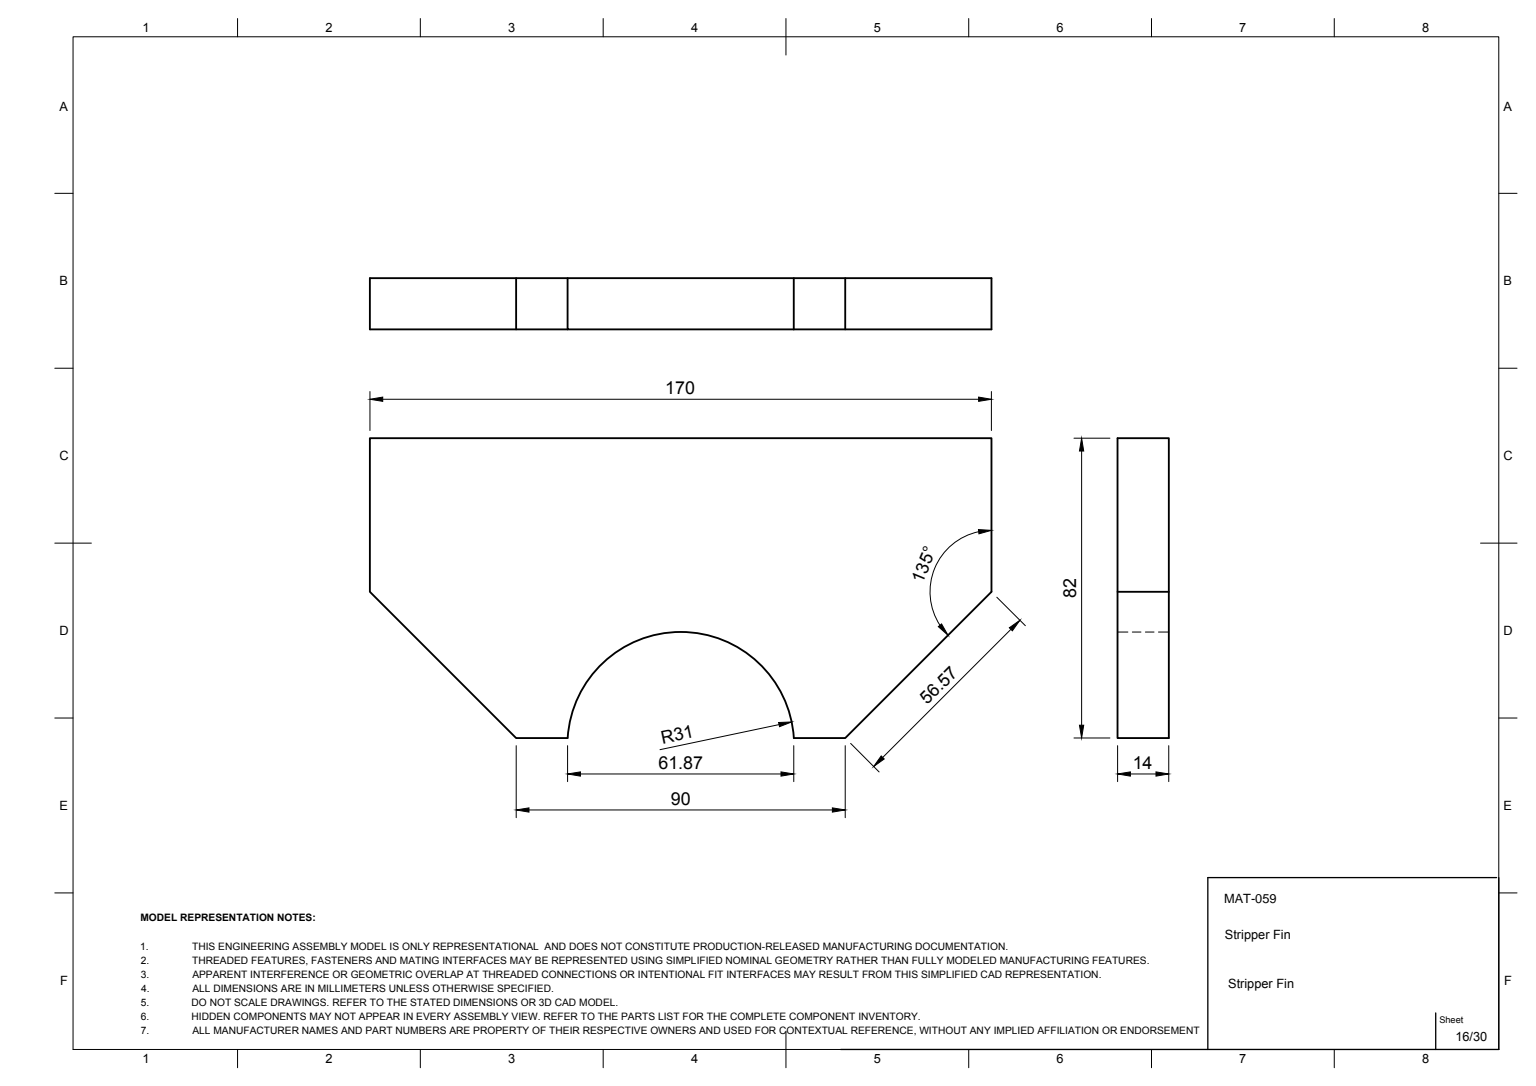
ISO-10303-21;
HEADER;
/* Generated by software containing ST-Developer
 * from STEP Tools, Inc. (www.steptools.com) 
 */

FILE_DESCRIPTION(
/* description */ ('', 'CAx-IF Rec.Pracs.---Representation and Presentation of Product Manufa
cturing Information (PMI)---4.0---2014-10-13'),
/* implementation_level */ '2;1');

FILE_NAME(
/* name */ 'Stripper Fin.step',
/* time_stamp */ '2026-10-28T23:00:48+01:00',
/* author */ (''),
/* organization */ (''),
/* preprocessor_version */ 'ST-DEVELOPER v20.2',
/* originating_system */ 'Autodesk Translation Framework v15.17.0.0',
/* authorisation */ '');

FILE_SCHEMA (('AP242_MANAGED_MODEL_BASED_3D_ENGINEERING_MIM_LF { 1 0 10303 442 2 1 4 }'));
ENDSEC;

DATA;
#10=MECHANICAL_DESIGN_GEOMETRIC_PRESENTATION_REPRESENTATION('',(#990),#61811);
#926=SHAPE_REPRESENTATION_RELATIONSHIP('SRR','None',#61985,#951);
#951=ADVANCED_BREP_SHAPE_REPRESENTATION('',(#1029),#61798);
#990=STYLED_ITEM('',(#62142),#1029);
#1029=MANIFOLD_SOLID_BREP('Body1',#33820);
#1365=CYLINDRICAL_SURFACE('',#35914,31.);
#3028=CIRCLE('',#35913,31.);
#3029=CIRCLE('',#35915,31.);
#5170=FACE_OUTER_BOUND('',#7276,.T.);
#5171=FACE_OUTER_BOUND('',#7277,.T.);
#5172=FACE_OUTER_BOUND('',#7278,.T.);
#5173=FACE_OUTER_BOUND('',#7279,.T.);
#5174=FACE_OUTER_BOUND('',#7280,.T.);
#5175=FACE_OUTER_BOUND('',#7281,.T.);
#5176=FACE_OUTER_BOUND('',#7282,.T.);
#5177=FACE_OUTER_BOUND('',#7283,.T.);
#5178=FACE_OUTER_BOUND('',#7284,.T.);
#5179=FACE_OUTER_BOUND('',#7285,.T.);
#7276=EDGE_LOOP('',(#26122,#26123,#26124,#26125));
#7277=EDGE_LOOP('',(#26126,#26127,#26128,#26129));
#7278=EDGE_LOOP('',(#26130,#26131,#26132,#26133,#26134,#26135,#26136,#26137));
#7279=EDGE_LOOP('',(#26138,#26139,#26140,#26141));
#7280=EDGE_LOOP('',(#26142,#26143,#26144,#26145,#26146,#26147,#26148,#26149));
#7281=EDGE_LOOP('',(#26150,#26151,#26152,#26153));
#7282=EDGE_LOOP('',(#26154,#26155,#26156,#26157));
#7283=EDGE_LOOP('',(#26158,#26159,#26160,#26161));
#7284=EDGE_LOOP('',(#26162,#26163,#26164,#26165));
#7285=EDGE_LOOP('',(#26166,#26167,#26168,#26169));
#9707=LINE('',#55749,#12254);
#9708=LINE('',#55751,#12255);
#9709=LINE('',#55753,#12256);
#9710=LINE('',#55754,#12257);
#9711=LINE('',#55757,#12258);
#9712=LINE('',#55759,#12259);
#9713=LINE('',#55760,#12260);
#9714=LINE('',#55763,#12261);
#9715=LINE('',#55765,#12262);
#9716=LINE('',#55767,#12263);
#9717=LINE('',#55771,#12264);
#9718=LINE('',#55772,#12265);
#9719=LINE('',#55775,#12266);
#9720=LINE('',#55777,#12267);
#9721=LINE('',#55781,#12268);
#9722=LINE('',#55782,#12269);
#9723=LINE('',#55784,#12270);
#9724=LINE('',#55786,#12271);
#9725=LINE('',#55787,#12272);
#9726=LINE('',#55789,#12273);
#9727=LINE('',#55791,#12274);
#9728=LINE('',#55793,#12275);
#12254=VECTOR('',#43125,10.);
#12255=VECTOR('',#43126,10.);
#12256=VECTOR('',#43127,10.);
#12257=VECTOR('',#43128,10.);
#12258=VECTOR('',#43131,10.);
#12259=VECTOR('',#43132,10.);
#12260=VECTOR('',#43133,10.);
#12261=VECTOR('',#43136,10.);
#12262=VECTOR('',#43137,10.);
#12263=VECTOR('',#43138,10.);
#12264=VECTOR('',#43141,10.);
#12265=VECTOR('',#43142,10.);
#12266=VECTOR('',#43145,10.);
#12267=VECTOR('',#43146,10.);
#12268=VECTOR('',#43151,10.);
#12269=VECTOR('',#43152,10.);
#12270=VECTOR('',#43153,10.);
#12271=VECTOR('',#43154,10.);
#12272=VECTOR('',#43155,10.);
#12273=VECTOR('',#43158,10.);
#12274=VECTOR('',#43161,10.);
#12275=VECTOR('',#43164,10.);
#14962=VERTEX_POINT('',#55747);
#14963=VERTEX_POINT('',#55748);
#14964=VERTEX_POINT('',#55750);
#14965=VERTEX_POINT('',#55752);
#14966=VERTEX_POINT('',#55756);
#14967=VERTEX_POINT('',#55758);
#14968=VERTEX_POINT('',#55762);
#14969=VERTEX_POINT('',#55764);
#14970=VERTEX_POINT('',#55766);
#14971=VERTEX_POINT('',#55768);
#14972=VERTEX_POINT('',#55770);
#14973=VERTEX_POINT('',#55774);
#14974=VERTEX_POINT('',#55776);
#14975=VERTEX_POINT('',#55780);
#14976=VERTEX_POINT('',#55783);
#14977=VERTEX_POINT('',#55785);
#18963=EDGE_CURVE('',#14962,#14963,#9707,.T.);
#18964=EDGE_CURVE('',#14964,#14962,#9708,.T.);
#18965=EDGE_CURVE('',#14965,#14964,#9709,.T.);
#18966=EDGE_CURVE('',#14963,#14965,#9710,.T.);
#18967=EDGE_CURVE('',#14965,#14966,#9711,.T.);
#18968=EDGE_CURVE('',#14967,#14966,#9712,.T.);
#18969=EDGE_CURVE('',#14967,#14963,#9713,.T.);
#18970=EDGE_CURVE('',#14964,#14968,#9714,.T.);
#18971=EDGE_CURVE('',#14969,#14968,#9715,.T.);
#18972=EDGE_CURVE('',#14970,#14969,#9716,.T.);
#18973=EDGE_CURVE('',#14970,#14971,#3028,.T.);
#18974=EDGE_CURVE('',#14972,#14971,#9717,.T.);
#18975=EDGE_CURVE('',#14966,#14972,#9718,.T.);
#18976=EDGE_CURVE('',#14971,#14973,#9719,.T.);
#18977=EDGE_CURVE('',#14974,#14970,#9720,.T.);
#18978=EDGE_CURVE('',#14973,#14974,#3029,.T.);
#18979=EDGE_CURVE('',#14975,#14967,#9721,.T.);
#18980=EDGE_CURVE('',#14973,#14975,#9722,.T.);
#18981=EDGE_CURVE('',#14976,#14974,#9723,.T.);
#18982=EDGE_CURVE('',#14977,#14976,#9724,.T.);
#18983=EDGE_CURVE('',#14977,#14962,#9725,.T.);
#18984=EDGE_CURVE('',#14976,#14969,#9726,.T.);
#18985=EDGE_CURVE('',#14972,#14975,#9727,.T.);
#18986=EDGE_CURVE('',#14968,#14977,#9728,.T.);
#26122=ORIENTED_EDGE('',*,*,#18963,.F.);
#26123=ORIENTED_EDGE('',*,*,#18964,.F.);
#26124=ORIENTED_EDGE('',*,*,#18965,.F.);
#26125=ORIENTED_EDGE('',*,*,#18966,.F.);
#26126=ORIENTED_EDGE('',*,*,#18966,.T.);
#26127=ORIENTED_EDGE('',*,*,#18967,.T.);
#26128=ORIENTED_EDGE('',*,*,#18968,.F.);
#26129=ORIENTED_EDGE('',*,*,#18969,.T.);
#26130=ORIENTED_EDGE('',*,*,#18965,.T.);
#26131=ORIENTED_EDGE('',*,*,#18970,.T.);
#26132=ORIENTED_EDGE('',*,*,#18971,.F.);
#26133=ORIENTED_EDGE('',*,*,#18972,.F.);
#26134=ORIENTED_EDGE('',*,*,#18973,.T.);
#26135=ORIENTED_EDGE('',*,*,#18974,.F.);
#26136=ORIENTED_EDGE('',*,*,#18975,.F.);
#26137=ORIENTED_EDGE('',*,*,#18967,.F.);
#26138=ORIENTED_EDGE('',*,*,#18976,.F.);
#26139=ORIENTED_EDGE('',*,*,#18973,.F.);
#26140=ORIENTED_EDGE('',*,*,#18977,.F.);
#26141=ORIENTED_EDGE('',*,*,#18978,.F.);
#26142=ORIENTED_EDGE('',*,*,#18963,.T.);
#26143=ORIENTED_EDGE('',*,*,#18969,.F.);
#26144=ORIENTED_EDGE('',*,*,#18979,.F.);
#26145=ORIENTED_EDGE('',*,*,#18980,.F.);
#26146=ORIENTED_EDGE('',*,*,#18978,.T.);
#26147=ORIENTED_EDGE('',*,*,#18981,.F.);
#26148=ORIENTED_EDGE('',*,*,#18982,.F.);
#26149=ORIENTED_EDGE('',*,*,#18983,.T.);
#26150=ORIENTED_EDGE('',*,*,#18977,.T.);
#26151=ORIENTED_EDGE('',*,*,#18972,.T.);
#26152=ORIENTED_EDGE('',*,*,#18984,.F.);
#26153=ORIENTED_EDGE('',*,*,#18981,.T.);
#26154=ORIENTED_EDGE('',*,*,#18976,.T.);
#26155=ORIENTED_EDGE('',*,*,#18980,.T.);
#26156=ORIENTED_EDGE('',*,*,#18985,.F.);
#26157=ORIENTED_EDGE('',*,*,#18974,.T.);
#26158=ORIENTED_EDGE('',*,*,#18982,.T.);
#26159=ORIENTED_EDGE('',*,*,#18984,.T.);
#26160=ORIENTED_EDGE('',*,*,#18971,.T.);
#26161=ORIENTED_EDGE('',*,*,#18986,.T.);
#26162=ORIENTED_EDGE('',*,*,#18975,.T.);
#26163=ORIENTED_EDGE('',*,*,#18985,.T.);
#26164=ORIENTED_EDGE('',*,*,#18979,.T.);
#26165=ORIENTED_EDGE('',*,*,#18968,.T.);
#26166=ORIENTED_EDGE('',*,*,#18964,.T.);
#26167=ORIENTED_EDGE('',*,*,#18983,.F.);
#26168=ORIENTED_EDGE('',*,*,#18986,.F.);
#26169=ORIENTED_EDGE('',*,*,#18970,.F.);
#31606=PLANE('',#35910);
#31607=PLANE('',#35911);
#31608=PLANE('',#35912);
#31609=PLANE('',#35916);
#31610=PLANE('',#35917);
#31611=PLANE('',#35918);
#31612=PLANE('',#35919);
#31613=PLANE('',#35920);
#31614=PLANE('',#35921);
#32851=ADVANCED_FACE('',(#5170),#31606,.F.);
#32852=ADVANCED_FACE('',(#5171),#31607,.F.);
#32853=ADVANCED_FACE('',(#5172),#31608,.T.);
#32854=ADVANCED_FACE('',(#5173),#1365,.F.);
#32855=ADVANCED_FACE('',(#5174),#31609,.T.);
#32856=ADVANCED_FACE('',(#5175),#31610,.T.);
#32857=ADVANCED_FACE('',(#5176),#31611,.T.);
#32858=ADVANCED_FACE('',(#5177),#31612,.T.);
#32859=ADVANCED_FACE('',(#5178),#31613,.T.);
#32860=ADVANCED_FACE('',(#5179),#31614,.T.);
#33820=CLOSED_SHELL('',(#32851,#32852,#32853,#32854,#32855,#32856,#32857,
#32858,#32859,#32860));
#35909=AXIS2_PLACEMENT_3D('',#55745,#43121,#43122);
#35910=AXIS2_PLACEMENT_3D('',#55746,#43123,#43124);
#35911=AXIS2_PLACEMENT_3D('',#55755,#43129,#43130);
#35912=AXIS2_PLACEMENT_3D('',#55761,#43134,#43135);
#35913=AXIS2_PLACEMENT_3D('',#55769,#43139,#43140);
#35914=AXIS2_PLACEMENT_3D('',#55773,#43143,#43144);
#35915=AXIS2_PLACEMENT_3D('',#55778,#43147,#43148);
#35916=AXIS2_PLACEMENT_3D('',#55779,#43149,#43150);
#35917=AXIS2_PLACEMENT_3D('',#55788,#43156,#43157);
#35918=AXIS2_PLACEMENT_3D('',#55790,#43159,#43160);
#35919=AXIS2_PLACEMENT_3D('',#55792,#43162,#43163);
#35920=AXIS2_PLACEMENT_3D('',#55794,#43165,#43166);
#35921=AXIS2_PLACEMENT_3D('',#55795,#43167,#43168);
#43121=DIRECTION('axis',(0.,0.,1.));
#43122=DIRECTION('refdir',(1.,0.,0.));
#43123=DIRECTION('center_axis',(-1.,-5.4480841862383E-16,3.82282413363175E-15));
#43124=DIRECTION('ref_axis',(-3.82282413363175E-15,3.2203325039861E-15,
-1.));
#43125=DIRECTION('',(3.82282413363175E-15,-3.2203325039861E-15,1.));
#43126=DIRECTION('',(5.44808418623818E-16,-1.,-3.2203325039861E-15));
#43127=DIRECTION('',(-3.82282413363175E-15,3.2203325039861E-15,-1.));
#43128=DIRECTION('',(-5.44808418623818E-16,1.,3.2203325039861E-15));
#43129=DIRECTION('center_axis',(-3.82282413363175E-15,3.2203325039861E-15,
-1.));
#43130=DIRECTION('ref_axis',(5.44808418623818E-16,-1.,-3.2203325039861E-15));
#43131=DIRECTION('',(-1.,-5.4480841862383E-16,3.82282413363175E-15));
#43132=DIRECTION('',(-5.44808418623818E-16,1.,3.2203325039861E-15));
#43133=DIRECTION('',(1.,5.4480841862383E-16,-3.82282413363175E-15));
#43134=DIRECTION('center_axis',(-5.44808418623818E-16,1.,3.2203325039861E-15));
#43135=DIRECTION('ref_axis',(1.,5.4480841862383E-16,-3.82282413363175E-15));
#43136=DIRECTION('',(-1.,-5.4480841862383E-16,3.82282413363175E-15));
#43137=DIRECTION('',(0.707106781186545,2.66235667850046E-15,-0.70710678118655));
#43138=DIRECTION('',(-3.82282413363175E-15,3.2203325039861E-15,-1.));
#43139=DIRECTION('center_axis',(5.44808418623818E-16,-1.,-3.2203325039861E-15));
#43140=DIRECTION('ref_axis',(3.82282413363175E-15,-3.2203325039861E-15,
1.));
#43141=DIRECTION('',(-3.82282413363175E-15,3.2203325039861E-15,-1.));
#43142=DIRECTION('',(-0.70710678118655,1.8918812239876E-15,-0.707106781186545));
#43143=DIRECTION('center_axis',(5.44808418623818E-16,-1.,-3.2203325039861E-15));
#43144=DIRECTION('ref_axis',(3.82282413363175E-15,-3.2203325039861E-15,
1.));
#43145=DIRECTION('',(5.44808418623818E-16,-1.,-3.2203325039861E-15));
#43146=DIRECTION('',(-5.44808418623818E-16,1.,3.2203325039861E-15));
#43147=DIRECTION('center_axis',(-5.44808418623818E-16,1.,3.2203325039861E-15));
#43148=DIRECTION('ref_axis',(3.82282413363175E-15,-3.2203325039861E-15,
1.));
#43149=DIRECTION('center_axis',(5.44808418623818E-16,-1.,-3.2203325039861E-15));
#43150=DIRECTION('ref_axis',(-1.,-5.4480841862383E-16,3.82282413363175E-15));
#43151=DIRECTION('',(0.70710678118655,-1.8918812239876E-15,0.707106781186545));
#43152=DIRECTION('',(3.82282413363175E-15,-3.2203325039861E-15,1.));
#43153=DIRECTION('',(3.82282413363175E-15,-3.2203325039861E-15,1.));
#43154=DIRECTION('',(-0.707106781186545,-2.66235667850046E-15,0.70710678118655));
#43155=DIRECTION('',(1.,5.4480841862383E-16,-3.82282413363175E-15));
#43156=DIRECTION('center_axis',(-1.,-5.4480841862383E-16,3.82282413363175E-15));
#43157=DIRECTION('ref_axis',(3.82282413363175E-15,-3.2203325039861E-15,
1.));
#43158=DIRECTION('',(-5.44808418623818E-16,1.,3.2203325039861E-15));
#43159=DIRECTION('center_axis',(-1.,-5.4480841862383E-16,3.82282413363175E-15));
#43160=DIRECTION('ref_axis',(3.82282413363175E-15,-3.2203325039861E-15,
1.));
#43161=DIRECTION('',(5.44808418623818E-16,-1.,-3.2203325039861E-15));
#43162=DIRECTION('center_axis',(-0.70710678118655,1.8918812239876E-15,-0.707106781186545));
#43163=DIRECTION('ref_axis',(5.44808418623818E-16,-1.,-3.2203325039861E-15));
#43164=DIRECTION('',(5.44808418623818E-16,-1.,-3.2203325039861E-15));
#43165=DIRECTION('center_axis',(-0.707106781186545,-2.66235667850046E-15,
0.70710678118655));
#43166=DIRECTION('ref_axis',(-5.44808418623818E-16,1.,3.2203325039861E-15));
#43167=DIRECTION('center_axis',(-3.82282413363175E-15,3.2203325039861E-15,
-1.));
#43168=DIRECTION('ref_axis',(5.44808418623818E-16,-1.,-3.2203325039861E-15));
#55745=CARTESIAN_POINT('',(0.,0.,0.));
#55746=CARTESIAN_POINT('Origin',(459.115917770968,-120.97200726879,530.000000551892));
#55747=CARTESIAN_POINT('',(459.115917770968,-134.97200726879,360.000000551892));
#55748=CARTESIAN_POINT('',(459.115917770968,-134.97200726879,530.000000551892));
#55749=CARTESIAN_POINT('',(459.115917770968,-134.97200726879,530.000000551892));
#55750=CARTESIAN_POINT('',(459.115917770968,-120.97200726879,360.000000551892));
#55751=CARTESIAN_POINT('',(459.115917770968,-124.47200726879,360.000000551892));
#55752=CARTESIAN_POINT('',(459.115917770968,-120.97200726879,530.000000551892));
#55753=CARTESIAN_POINT('',(459.115917770968,-120.97200726879,530.000000551892));
#55754=CARTESIAN_POINT('',(459.115917770968,-124.47200726879,530.000000551892));
#55755=CARTESIAN_POINT('Origin',(439.615917770968,-127.97200726879,530.000000551892));
#55756=CARTESIAN_POINT('',(417.115917770968,-120.97200726879,530.000000551893));
#55757=CARTESIAN_POINT('',(405.115917770968,-120.97200726879,530.000000551893));
#55758=CARTESIAN_POINT('',(417.115917770968,-134.97200726879,530.000000551893));
#55759=CARTESIAN_POINT('',(417.115917770968,-127.97200726879,530.000000551893));
#55760=CARTESIAN_POINT('',(405.115917770968,-134.97200726879,530.000000551893));
#55761=CARTESIAN_POINT('Origin',(405.115917770968,-120.97200726879,530.000000551893));
#55762=CARTESIAN_POINT('',(417.115917770967,-120.97200726879,360.000000551892));
#55763=CARTESIAN_POINT('',(422.365917770967,-120.97200726879,360.000000551892));
#55764=CARTESIAN_POINT('',(377.115917770967,-120.97200726879,400.000000551893));
#55765=CARTESIAN_POINT('',(361.615917770967,-120.97200726879,415.500000551893));
#55766=CARTESIAN_POINT('',(377.115917770967,-120.97200726879,414.064583955377));
#55767=CARTESIAN_POINT('',(377.115917770968,-120.97200726879,530.000000551893));
#55768=CARTESIAN_POINT('',(377.115917770967,-120.97200726879,475.935417148409));
#55769=CARTESIAN_POINT('Origin',(375.115917770968,-120.97200726879,445.000000551893));
#55770=CARTESIAN_POINT('',(377.115917770968,-120.97200726879,490.000000551893));
#55771=CARTESIAN_POINT('',(377.115917770968,-120.97200726879,530.000000551893));
#55772=CARTESIAN_POINT('',(404.115917770968,-120.97200726879,517.000000551893));
#55773=CARTESIAN_POINT('Origin',(375.115917770968,-120.97200726879,445.000000551893));
#55774=CARTESIAN_POINT('',(377.115917770967,-134.97200726879,475.935417148409));
#55775=CARTESIAN_POINT('',(377.115917770967,-120.97200726879,475.935417148409));
#55776=CARTESIAN_POINT('',(377.115917770967,-134.97200726879,414.064583955377));
#55777=CARTESIAN_POINT('',(377.115917770967,-120.97200726879,414.064583955377));
#55778=CARTESIAN_POINT('Origin',(375.115917770968,-134.97200726879,445.000000551893));
#55779=CARTESIAN_POINT('Origin',(474.115917770968,-134.97200726879,530.000000551892));
#55780=CARTESIAN_POINT('',(377.115917770968,-134.97200726879,490.000000551893));
#55781=CARTESIAN_POINT('',(421.365917770968,-134.97200726879,534.250000551893));
#55782=CARTESIAN_POINT('',(377.115917770967,-134.97200726879,360.000000551893));
#55783=CARTESIAN_POINT('',(377.115917770967,-134.97200726879,400.000000551893));
#55784=CARTESIAN_POINT('',(377.115917770967,-134.97200726879,360.000000551893));
#55785=CARTESIAN_POINT('',(417.115917770967,-134.97200726879,360.000000551892));
#55786=CARTESIAN_POINT('',(378.865917770968,-134.97200726879,398.250000551893));
#55787=CARTESIAN_POINT('',(456.865917770968,-134.97200726879,360.000000551892));
#55788=CARTESIAN_POINT('Origin',(377.115917770967,-127.97200726879,445.000000551893));
#55789=CARTESIAN_POINT('',(377.115917770967,-127.97200726879,400.000000551893));
#55790=CARTESIAN_POINT('Origin',(377.115917770967,-127.97200726879,445.000000551893));
#55791=CARTESIAN_POINT('',(377.115917770968,-127.97200726879,490.000000551893));
#55792=CARTESIAN_POINT('Origin',(397.115917770967,-127.97200726879,380.000000551893));
#55793=CARTESIAN_POINT('',(417.115917770967,-127.97200726879,360.000000551892));
#55794=CARTESIAN_POINT('Origin',(397.115917770968,-127.97200726879,510.000000551893));
#55795=CARTESIAN_POINT('Origin',(439.615917770967,-127.97200726879,360.000000551892));
#61767=UNCERTAINTY_MEASURE_WITH_UNIT(LENGTH_MEASURE(0.01),#61812,
'DISTANCE_ACCURACY_VALUE',
'Maximum model space distance between geometric entities at asserted c
onnectivities');
#61780=UNCERTAINTY_MEASURE_WITH_UNIT(LENGTH_MEASURE(0.01),#61812,
'DISTANCE_ACCURACY_VALUE',
'Maximum model space distance between geometric entities at asserted c
onnectivities');
#61798=(
GEOMETRIC_REPRESENTATION_CONTEXT(3)
GLOBAL_UNCERTAINTY_ASSIGNED_CONTEXT((#61767))
GLOBAL_UNIT_ASSIGNED_CONTEXT((#61812,#61814,#61815))
REPRESENTATION_CONTEXT('','3D')
);
#61811=(
GEOMETRIC_REPRESENTATION_CONTEXT(3)
GLOBAL_UNCERTAINTY_ASSIGNED_CONTEXT((#61780))
GLOBAL_UNIT_ASSIGNED_CONTEXT((#61812,#61814,#61815))
REPRESENTATION_CONTEXT('','3D')
);
#61812=(
LENGTH_UNIT()
NAMED_UNIT(*)
SI_UNIT(.MILLI.,.METRE.)
);
#61814=(
NAMED_UNIT(*)
PLANE_ANGLE_UNIT()
SI_UNIT($,.RADIAN.)
);
#61815=(
NAMED_UNIT(*)
SI_UNIT($,.STERADIAN.)
SOLID_ANGLE_UNIT()
);
#61833=SHAPE_DEFINITION_REPRESENTATION(#61863,#61985);
#61863=PRODUCT_DEFINITION_SHAPE('',$,#62016);
#61985=SHAPE_REPRESENTATION('',(#35909),#61798);
#61998=PRODUCT_DEFINITION_CONTEXT('part definition',#62090,'design');
#62016=PRODUCT_DEFINITION('Stripper Fin','Stripper Fin',#62046,#61998);
#62046=PRODUCT_DEFINITION_FORMATION('',$,#62109);
#62090=APPLICATION_CONTEXT('Managed model based 3d engineering');
#62091=PRODUCT_CONTEXT('part definition',#62090,'mechanical');
#62109=PRODUCT('Stripper Fin','Stripper Fin',$,(#62091));
#62136=COLOUR_RGB('Light Blue',0.38,0.62,0.78);
#62137=FILL_AREA_STYLE_COLOUR('',#62136);
#62138=FILL_AREA_STYLE('',(#62137));
#62139=SURFACE_STYLE_FILL_AREA(#62138);
#62140=SURFACE_SIDE_STYLE('',(#62139));
#62141=SURFACE_STYLE_USAGE(.BOTH.,#62140);
#62142=PRESENTATION_STYLE_ASSIGNMENT((#62141));
ENDSEC;
END-ISO-10303-21;
